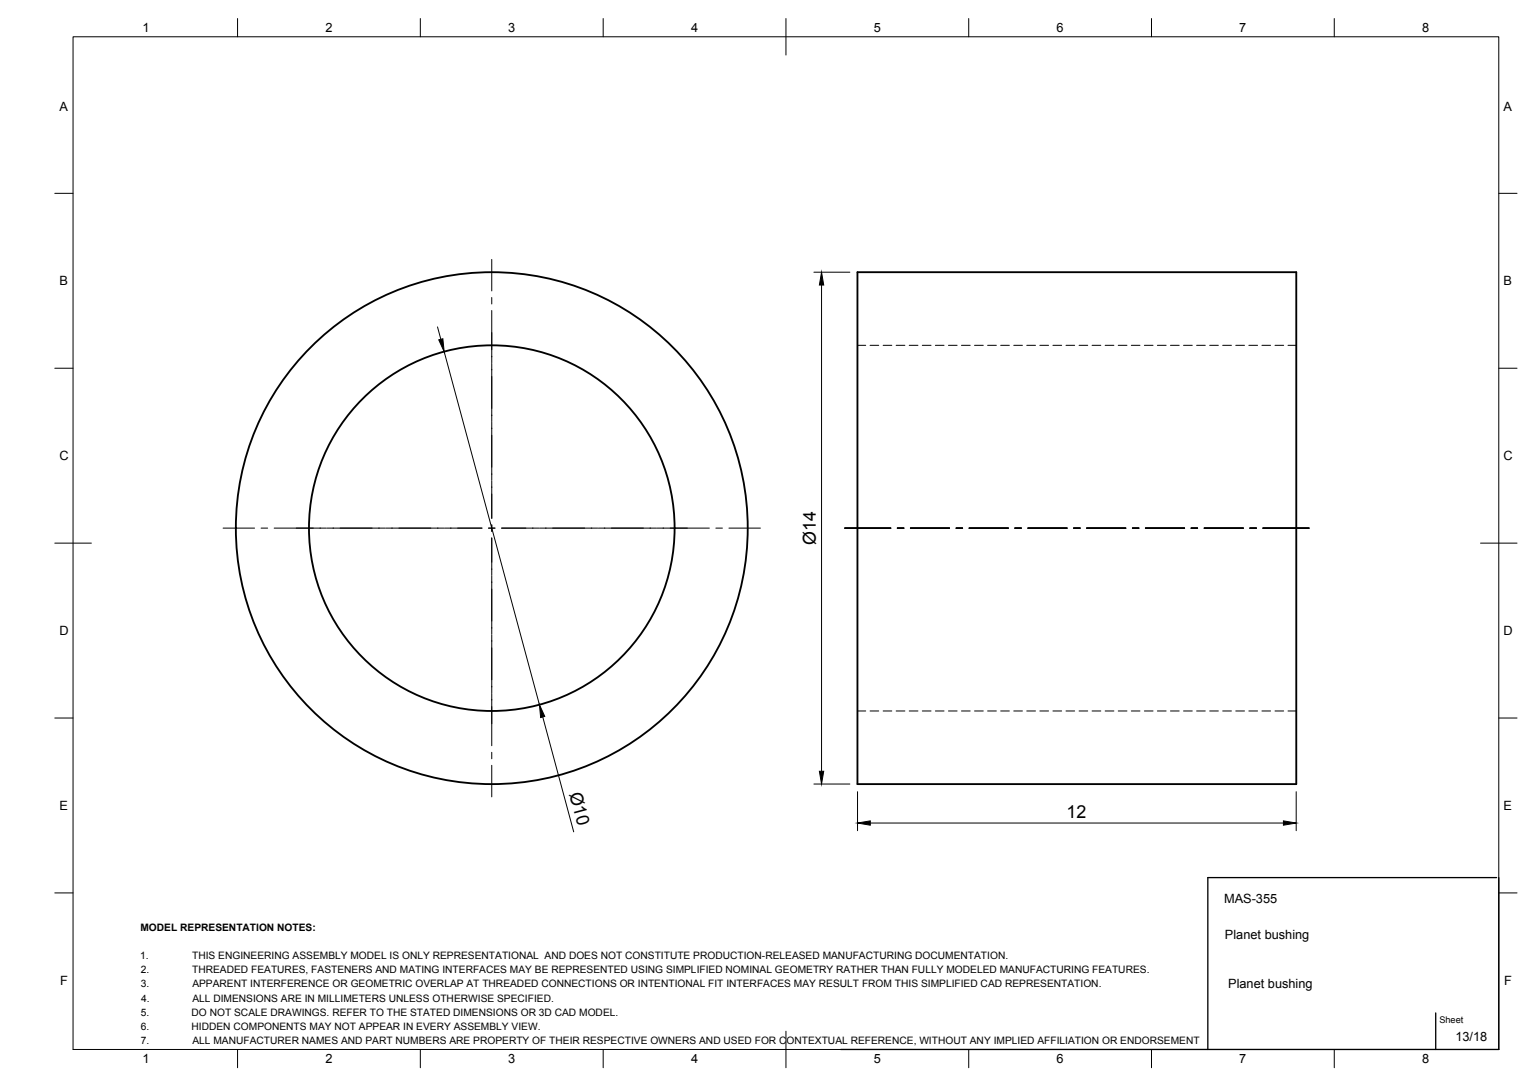
ISO-10303-21;
HEADER;
/* Generated by software containing ST-Developer
 * from STEP Tools, Inc. (www.steptools.com) 
 */

FILE_DESCRIPTION(
/* description */ ('Independent two-stage fixed-ring planetary gearbox,24/24/72 teeth,mod
ule2,20deg involutes,three planets per stage,4:1 x4:1=16:1. Native cut
-space/fillet/pattern tooth profiles derived from reusable gear blanks
; shared sun/planet/ring/carrier parts across both stages. Captured br
onze-journal input/carriers, headed retained planet pins, keyed inters
tage drive and modular keyed output interface. Native ideal gear links
; no torque, precision grade, production backlash/fits, lubrication, s
peed or life rating.'),
/* implementation_level */ '2;1');

FILE_NAME(
/* name */ 'Planet bushing.step',
/* time_stamp */ '2026-11-08T19:10:00-08:00',
/* author */ (''),
/* organization */ (''),
/* preprocessor_version */ 'ST-DEVELOPER v20.2',
/* originating_system */ 'Autodesk Translation Framework v15.17.0.0',
/* authorisation */ '');

FILE_SCHEMA (('AUTOMOTIVE_DESIGN { 1 0 10303 214 3 1 1 }'));
ENDSEC;

DATA;
#10=MECHANICAL_DESIGN_GEOMETRIC_PRESENTATION_REPRESENTATION('',(#1173),#259224);
#1133=SHAPE_REPRESENTATION_RELATIONSHIP('SRR','None',#259380,#1153);
#1153=ADVANCED_BREP_SHAPE_REPRESENTATION('',(#1193),#259214);
#1173=STYLED_ITEM('',(#259485),#1193);
#1193=MANIFOLD_SOLID_BREP('Body1',#25160);
#1305=FACE_BOUND('',#4394,.T.);
#1306=FACE_BOUND('',#4396,.T.);
#1661=PLANE('',#27090);
#1662=PLANE('',#27091);
#2943=FACE_OUTER_BOUND('',#4391,.T.);
#2944=FACE_OUTER_BOUND('',#4392,.T.);
#2945=FACE_OUTER_BOUND('',#4393,.T.);
#2946=FACE_OUTER_BOUND('',#4395,.T.);
#4391=EDGE_LOOP('',(#22622,#22623,#22624,#22625));
#4392=EDGE_LOOP('',(#22626,#22627,#22628,#22629));
#4393=EDGE_LOOP('',(#22630));
#4394=EDGE_LOOP('',(#22631));
#4395=EDGE_LOOP('',(#22632));
#4396=EDGE_LOOP('',(#22633));
#5341=CIRCLE('',#27085,5.);
#5342=CIRCLE('',#27086,5.);
#5343=CIRCLE('',#27088,7.);
#5344=CIRCLE('',#27089,7.);
#7756=LINE('',#255933,#8941);
#7757=LINE('',#255939,#8942);
#8941=VECTOR('',#31813,5.);
#8942=VECTOR('',#31820,7.);
#11445=VERTEX_POINT('',#255930);
#11446=VERTEX_POINT('',#255932);
#11447=VERTEX_POINT('',#255936);
#11448=VERTEX_POINT('',#255938);
#15196=EDGE_CURVE('',#11445,#11445,#5341,.T.);
#15197=EDGE_CURVE('',#11445,#11446,#7756,.T.);
#15198=EDGE_CURVE('',#11446,#11446,#5342,.T.);
#15199=EDGE_CURVE('',#11447,#11447,#5343,.T.);
#15200=EDGE_CURVE('',#11447,#11448,#7757,.T.);
#15201=EDGE_CURVE('',#11448,#11448,#5344,.T.);
#22622=ORIENTED_EDGE('',*,*,#15196,.F.);
#22623=ORIENTED_EDGE('',*,*,#15197,.T.);
#22624=ORIENTED_EDGE('',*,*,#15198,.T.);
#22625=ORIENTED_EDGE('',*,*,#15197,.F.);
#22626=ORIENTED_EDGE('',*,*,#15199,.F.);
#22627=ORIENTED_EDGE('',*,*,#15200,.T.);
#22628=ORIENTED_EDGE('',*,*,#15201,.T.);
#22629=ORIENTED_EDGE('',*,*,#15200,.F.);
#22630=ORIENTED_EDGE('',*,*,#15199,.T.);
#22631=ORIENTED_EDGE('',*,*,#15196,.T.);
#22632=ORIENTED_EDGE('',*,*,#15201,.F.);
#22633=ORIENTED_EDGE('',*,*,#15198,.F.);
#23742=CYLINDRICAL_SURFACE('',#27084,5.);
#23743=CYLINDRICAL_SURFACE('',#27087,7.);
#25049=ADVANCED_FACE('',(#2943),#23742,.F.);
#25050=ADVANCED_FACE('',(#2944),#23743,.T.);
#25051=ADVANCED_FACE('',(#2945,#1305),#1661,.T.);
#25052=ADVANCED_FACE('',(#2946,#1306),#1662,.F.);
#25160=CLOSED_SHELL('',(#25049,#25050,#25051,#25052));
#27083=AXIS2_PLACEMENT_3D('',#255928,#31807,#31808);
#27084=AXIS2_PLACEMENT_3D('',#255929,#31809,#31810);
#27085=AXIS2_PLACEMENT_3D('',#255931,#31811,#31812);
#27086=AXIS2_PLACEMENT_3D('',#255934,#31814,#31815);
#27087=AXIS2_PLACEMENT_3D('',#255935,#31816,#31817);
#27088=AXIS2_PLACEMENT_3D('',#255937,#31818,#31819);
#27089=AXIS2_PLACEMENT_3D('',#255940,#31821,#31822);
#27090=AXIS2_PLACEMENT_3D('',#255941,#31823,#31824);
#27091=AXIS2_PLACEMENT_3D('',#255942,#31825,#31826);
#31807=DIRECTION('axis',(0.,0.,1.));
#31808=DIRECTION('refdir',(1.,0.,0.));
#31809=DIRECTION('center_axis',(0.,0.,1.));
#31810=DIRECTION('ref_axis',(1.,0.,0.));
#31811=DIRECTION('center_axis',(0.,0.,-1.));
#31812=DIRECTION('ref_axis',(1.,0.,0.));
#31813=DIRECTION('',(0.,0.,-1.));
#31814=DIRECTION('center_axis',(0.,0.,-1.));
#31815=DIRECTION('ref_axis',(1.,0.,0.));
#31816=DIRECTION('center_axis',(0.,0.,1.));
#31817=DIRECTION('ref_axis',(1.,0.,0.));
#31818=DIRECTION('center_axis',(0.,0.,1.));
#31819=DIRECTION('ref_axis',(1.,0.,0.));
#31820=DIRECTION('',(0.,0.,-1.));
#31821=DIRECTION('center_axis',(0.,0.,1.));
#31822=DIRECTION('ref_axis',(1.,0.,0.));
#31823=DIRECTION('center_axis',(0.,0.,1.));
#31824=DIRECTION('ref_axis',(1.,0.,0.));
#31825=DIRECTION('center_axis',(0.,0.,1.));
#31826=DIRECTION('ref_axis',(1.,0.,0.));
#255928=CARTESIAN_POINT('',(0.,0.,0.));
#255929=CARTESIAN_POINT('Origin',(0.,0.,0.));
#255930=CARTESIAN_POINT('',(-5.,-6.12323399573677E-16,12.));
#255931=CARTESIAN_POINT('Origin',(0.,0.,12.));
#255932=CARTESIAN_POINT('',(-5.,-6.12323399573677E-16,0.));
#255933=CARTESIAN_POINT('',(-5.,-6.12323399573677E-16,0.));
#255934=CARTESIAN_POINT('Origin',(0.,0.,0.));
#255935=CARTESIAN_POINT('Origin',(0.,0.,0.));
#255936=CARTESIAN_POINT('',(-7.,-8.57252759403147E-16,12.));
#255937=CARTESIAN_POINT('Origin',(0.,0.,12.));
#255938=CARTESIAN_POINT('',(-7.,-8.57252759403147E-16,0.));
#255939=CARTESIAN_POINT('',(-7.,-8.57252759403147E-16,0.));
#255940=CARTESIAN_POINT('Origin',(0.,0.,0.));
#255941=CARTESIAN_POINT('Origin',(0.,0.,12.));
#255942=CARTESIAN_POINT('Origin',(0.,0.,0.));
#259192=UNCERTAINTY_MEASURE_WITH_UNIT(LENGTH_MEASURE(0.01),#259225,
'DISTANCE_ACCURACY_VALUE',
'Maximum model space distance between geometric entities at asserted c
onnectivities');
#259202=UNCERTAINTY_MEASURE_WITH_UNIT(LENGTH_MEASURE(0.01),#259225,
'DISTANCE_ACCURACY_VALUE',
'Maximum model space distance between geometric entities at asserted c
onnectivities');
#259214=(
GEOMETRIC_REPRESENTATION_CONTEXT(3)
GLOBAL_UNCERTAINTY_ASSIGNED_CONTEXT((#259192))
GLOBAL_UNIT_ASSIGNED_CONTEXT((#259225,#259227,#259228))
REPRESENTATION_CONTEXT('','3D')
);
#259224=(
GEOMETRIC_REPRESENTATION_CONTEXT(3)
GLOBAL_UNCERTAINTY_ASSIGNED_CONTEXT((#259202))
GLOBAL_UNIT_ASSIGNED_CONTEXT((#259225,#259227,#259228))
REPRESENTATION_CONTEXT('','3D')
);
#259225=(
LENGTH_UNIT()
NAMED_UNIT(*)
SI_UNIT(.MILLI.,.METRE.)
);
#259227=(
NAMED_UNIT(*)
PLANE_ANGLE_UNIT()
SI_UNIT($,.RADIAN.)
);
#259228=(
NAMED_UNIT(*)
SI_UNIT($,.STERADIAN.)
SOLID_ANGLE_UNIT()
);
#259240=SHAPE_DEFINITION_REPRESENTATION(#259261,#259380);
#259261=PRODUCT_DEFINITION_SHAPE('',$,#259402);
#259380=SHAPE_REPRESENTATION('',(#27083),#259214);
#259390=PRODUCT_DEFINITION_CONTEXT('part definition',#259455,'design');
#259402=PRODUCT_DEFINITION('Planet bushing','Planet bushing',#259423,#259390);
#259423=PRODUCT_DEFINITION_FORMATION('',$,#259468);
#259455=APPLICATION_CONTEXT(
'Core Data for Automotive Mechanical Design Process');
#259456=PRODUCT_CONTEXT('part definition',#259455,'mechanical');
#259468=PRODUCT('Planet bushing','Planet bushing',$,(#259456));
#259485=PRESENTATION_STYLE_ASSIGNMENT((#259500));
#259500=SURFACE_STYLE_USAGE(.BOTH.,#259515);
#259515=SURFACE_SIDE_STYLE('',(#259530));
#259530=SURFACE_STYLE_FILL_AREA(#259545);
#259545=FILL_AREA_STYLE('Bearing light gray',(#259560));
#259560=FILL_AREA_STYLE_COLOUR('Bearing light gray',#259575);
#259575=COLOUR_RGB('Bearing light gray',0.725490196078431,0.752941176470588,
0.792156862745098);
ENDSEC;
END-ISO-10303-21;
